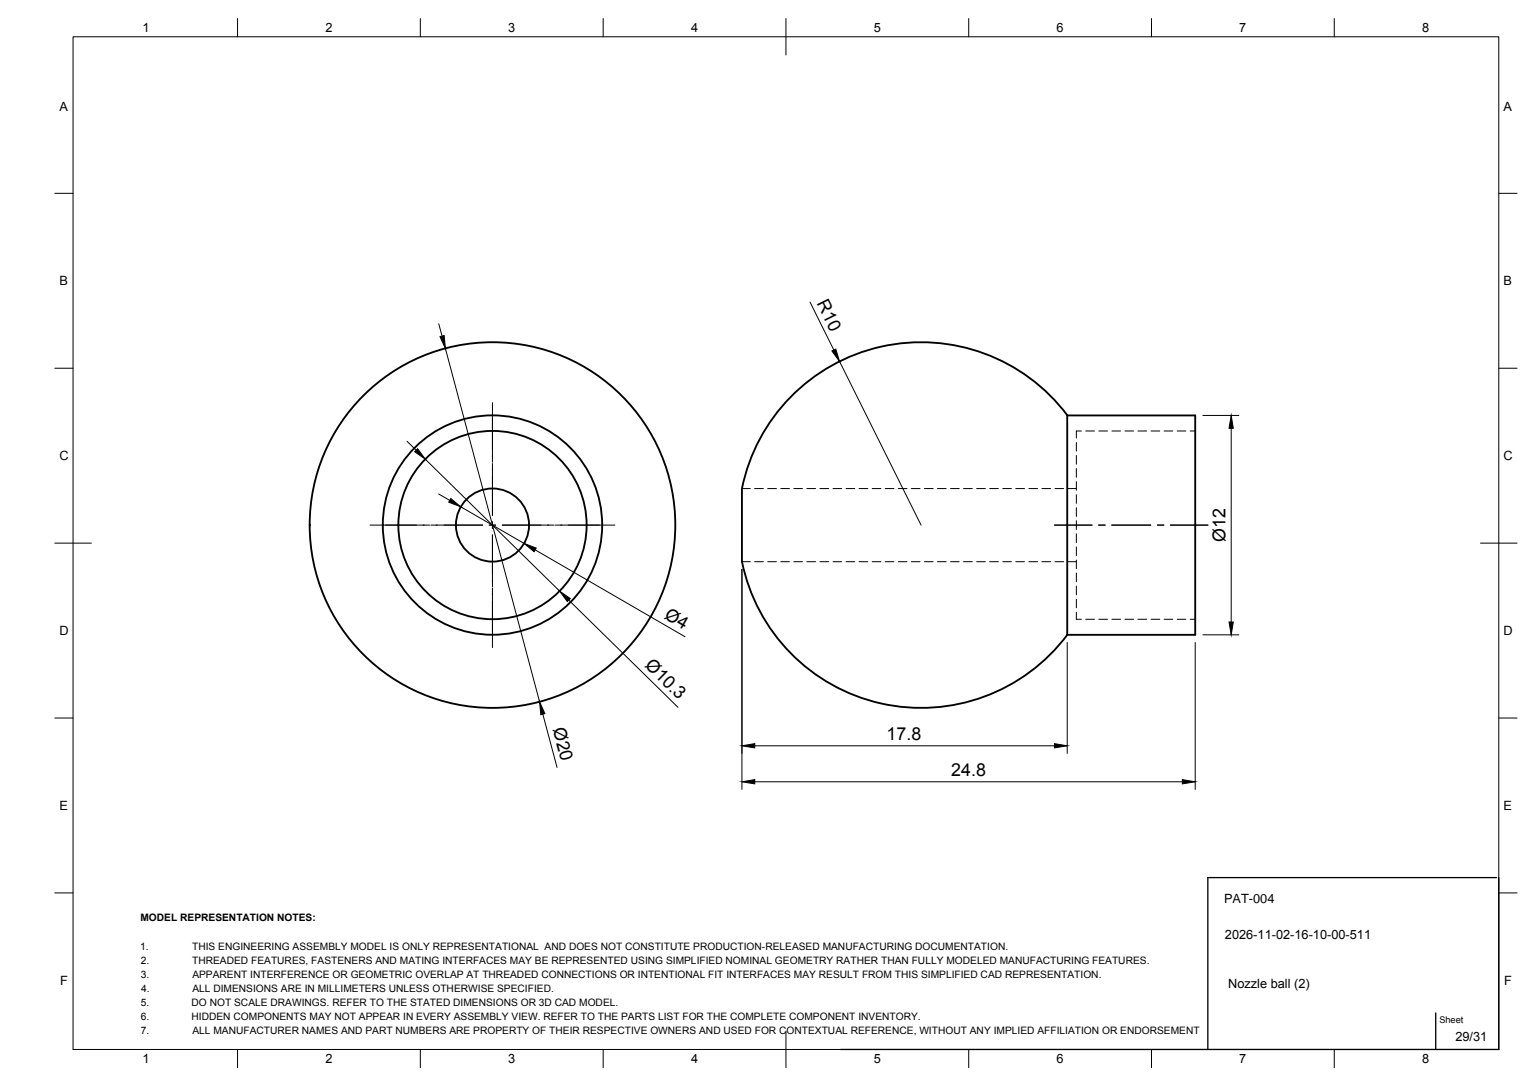
ISO-10303-21;
HEADER;
/* Generated by software containing ST-Developer
 * from STEP Tools, Inc. (www.steptools.com) 
 */

FILE_DESCRIPTION(
/* description */ ('Air blow-off nozzle station'),
/* implementation_level */ '2;1');

FILE_NAME(
/* name */ 'Nozzle ball (2).step',
/* time_stamp */ '2026-10-27T10:53:54-07:00',
/* author */ (''),
/* organization */ (''),
/* preprocessor_version */ 'ST-DEVELOPER v20.2',
/* originating_system */ 'Autodesk Translation Framework v15.17.0.0',
/* authorisation */ '');

FILE_SCHEMA (('AUTOMOTIVE_DESIGN { 1 0 10303 214 3 1 1 }'));
ENDSEC;

DATA;
#10=MECHANICAL_DESIGN_GEOMETRIC_PRESENTATION_REPRESENTATION('',(#257),#7897);
#170=SPHERICAL_SURFACE('',#4988,1.);
#207=SHAPE_REPRESENTATION_RELATIONSHIP('SRR','None',#8024,#232);
#232=ADVANCED_BREP_SHAPE_REPRESENTATION('',(#280),#7891);
#257=STYLED_ITEM('',(#8234),#280);
#280=MANIFOLD_SOLID_BREP('Body1',#4308);
#353=FACE_BOUND('',#1083,.T.);
#354=FACE_BOUND('',#1087,.T.);
#355=FACE_BOUND('',#1089,.T.);
#356=FACE_BOUND('',#1090,.T.);
#518=PLANE('',#4980);
#519=PLANE('',#4987);
#757=FACE_OUTER_BOUND('',#1081,.T.);
#758=FACE_OUTER_BOUND('',#1082,.T.);
#759=FACE_OUTER_BOUND('',#1084,.T.);
#760=FACE_OUTER_BOUND('',#1085,.T.);
#761=FACE_OUTER_BOUND('',#1086,.T.);
#762=FACE_OUTER_BOUND('',#1088,.T.);
#1081=EDGE_LOOP('',(#3825,#3826,#3827,#3828));
#1082=EDGE_LOOP('',(#3829));
#1083=EDGE_LOOP('',(#3830));
#1084=EDGE_LOOP('',(#3831,#3832,#3833,#3834));
#1085=EDGE_LOOP('',(#3835,#3836,#3837,#3838));
#1086=EDGE_LOOP('',(#3839));
#1087=EDGE_LOOP('',(#3840));
#1088=EDGE_LOOP('',(#3841,#3842));
#1089=EDGE_LOOP('',(#3843));
#1090=EDGE_LOOP('',(#3844));
#1458=LINE('',#7663,#1812);
#1459=LINE('',#7670,#1813);
#1460=LINE('',#7676,#1814);
#1812=VECTOR('',#6172,0.515);
#1813=VECTOR('',#6181,0.2);
#1814=VECTOR('',#6188,0.6);
#1974=CIRCLE('',#4978,0.515);
#1975=CIRCLE('',#4979,0.515);
#1976=CIRCLE('',#4981,0.2);
#1977=CIRCLE('',#4983,0.2);
#1978=CIRCLE('',#4985,0.6);
#1979=CIRCLE('',#4986,0.6);
#1980=CIRCLE('',#4989,1.);
#2320=VERTEX_POINT('',#7660);
#2321=VERTEX_POINT('',#7662);
#2322=VERTEX_POINT('',#7666);
#2323=VERTEX_POINT('',#7669);
#2324=VERTEX_POINT('',#7673);
#2325=VERTEX_POINT('',#7675);
#2326=VERTEX_POINT('',#7680);
#2327=VERTEX_POINT('',#7681);
#2830=EDGE_CURVE('',#2320,#2320,#1974,.T.);
#2831=EDGE_CURVE('',#2320,#2321,#1458,.T.);
#2832=EDGE_CURVE('',#2321,#2321,#1975,.T.);
#2833=EDGE_CURVE('',#2322,#2322,#1976,.T.);
#2834=EDGE_CURVE('',#2322,#2323,#1459,.T.);
#2835=EDGE_CURVE('',#2323,#2323,#1977,.T.);
#2836=EDGE_CURVE('',#2324,#2324,#1978,.T.);
#2837=EDGE_CURVE('',#2324,#2325,#1460,.T.);
#2838=EDGE_CURVE('',#2325,#2325,#1979,.T.);
#2839=EDGE_CURVE('',#2326,#2327,#1980,.T.);
#3825=ORIENTED_EDGE('',*,*,#2830,.F.);
#3826=ORIENTED_EDGE('',*,*,#2831,.T.);
#3827=ORIENTED_EDGE('',*,*,#2832,.T.);
#3828=ORIENTED_EDGE('',*,*,#2831,.F.);
#3829=ORIENTED_EDGE('',*,*,#2832,.F.);
#3830=ORIENTED_EDGE('',*,*,#2833,.F.);
#3831=ORIENTED_EDGE('',*,*,#2833,.T.);
#3832=ORIENTED_EDGE('',*,*,#2834,.T.);
#3833=ORIENTED_EDGE('',*,*,#2835,.F.);
#3834=ORIENTED_EDGE('',*,*,#2834,.F.);
#3835=ORIENTED_EDGE('',*,*,#2836,.F.);
#3836=ORIENTED_EDGE('',*,*,#2837,.T.);
#3837=ORIENTED_EDGE('',*,*,#2838,.T.);
#3838=ORIENTED_EDGE('',*,*,#2837,.F.);
#3839=ORIENTED_EDGE('',*,*,#2838,.F.);
#3840=ORIENTED_EDGE('',*,*,#2830,.T.);
#3841=ORIENTED_EDGE('',*,*,#2839,.T.);
#3842=ORIENTED_EDGE('',*,*,#2839,.F.);
#3843=ORIENTED_EDGE('',*,*,#2835,.T.);
#3844=ORIENTED_EDGE('',*,*,#2836,.T.);
#4014=CYLINDRICAL_SURFACE('',#4977,0.515);
#4015=CYLINDRICAL_SURFACE('',#4982,0.2);
#4016=CYLINDRICAL_SURFACE('',#4984,0.6);
#4247=ADVANCED_FACE('',(#757),#4014,.F.);
#4248=ADVANCED_FACE('',(#758,#353),#518,.F.);
#4249=ADVANCED_FACE('',(#759),#4015,.F.);
#4250=ADVANCED_FACE('',(#760),#4016,.T.);
#4251=ADVANCED_FACE('',(#761,#354),#519,.F.);
#4252=ADVANCED_FACE('',(#762,#355,#356),#170,.T.);
#4308=CLOSED_SHELL('',(#4247,#4248,#4249,#4250,#4251,#4252));
#4976=AXIS2_PLACEMENT_3D('',#7658,#6166,#6167);
#4977=AXIS2_PLACEMENT_3D('',#7659,#6168,#6169);
#4978=AXIS2_PLACEMENT_3D('',#7661,#6170,#6171);
#4979=AXIS2_PLACEMENT_3D('',#7664,#6173,#6174);
#4980=AXIS2_PLACEMENT_3D('',#7665,#6175,#6176);
#4981=AXIS2_PLACEMENT_3D('',#7667,#6177,#6178);
#4982=AXIS2_PLACEMENT_3D('',#7668,#6179,#6180);
#4983=AXIS2_PLACEMENT_3D('',#7671,#6182,#6183);
#4984=AXIS2_PLACEMENT_3D('',#7672,#6184,#6185);
#4985=AXIS2_PLACEMENT_3D('',#7674,#6186,#6187);
#4986=AXIS2_PLACEMENT_3D('',#7677,#6189,#6190);
#4987=AXIS2_PLACEMENT_3D('',#7678,#6191,#6192);
#4988=AXIS2_PLACEMENT_3D('',#7679,#6193,#6194);
#4989=AXIS2_PLACEMENT_3D('',#7682,#6195,#6196);
#6166=DIRECTION('axis',(0.,0.,1.));
#6167=DIRECTION('refdir',(1.,0.,0.));
#6168=DIRECTION('center_axis',(0.,1.,0.));
#6169=DIRECTION('ref_axis',(1.,0.,0.));
#6170=DIRECTION('center_axis',(0.,1.,0.));
#6171=DIRECTION('ref_axis',(1.,0.,0.));
#6172=DIRECTION('',(0.,1.,0.));
#6173=DIRECTION('center_axis',(0.,1.,0.));
#6174=DIRECTION('ref_axis',(1.,0.,0.));
#6175=DIRECTION('center_axis',(0.,1.,0.));
#6176=DIRECTION('ref_axis',(1.,0.,0.));
#6177=DIRECTION('center_axis',(0.,-1.,0.));
#6178=DIRECTION('ref_axis',(1.,0.,0.));
#6179=DIRECTION('center_axis',(0.,1.,0.));
#6180=DIRECTION('ref_axis',(1.,0.,0.));
#6181=DIRECTION('',(0.,1.,0.));
#6182=DIRECTION('center_axis',(0.,-1.,0.));
#6183=DIRECTION('ref_axis',(1.,-1.11022302462516E-15,0.));
#6184=DIRECTION('center_axis',(0.,1.,0.));
#6185=DIRECTION('ref_axis',(1.,0.,0.));
#6186=DIRECTION('center_axis',(0.,1.,0.));
#6187=DIRECTION('ref_axis',(1.,0.,0.));
#6188=DIRECTION('',(0.,-1.,0.));
#6189=DIRECTION('center_axis',(0.,1.,0.));
#6190=DIRECTION('ref_axis',(1.,0.,0.));
#6191=DIRECTION('center_axis',(0.,1.,0.));
#6192=DIRECTION('ref_axis',(1.,0.,0.));
#6193=DIRECTION('center_axis',(0.,0.,1.));
#6194=DIRECTION('ref_axis',(1.,0.,0.));
#6195=DIRECTION('center_axis',(0.,-1.,0.));
#6196=DIRECTION('ref_axis',(-1.,0.,0.));
#7658=CARTESIAN_POINT('',(0.,0.,0.));
#7659=CARTESIAN_POINT('Origin',(3.,-3.6,23.));
#7660=CARTESIAN_POINT('',(2.485,-3.5,23.));
#7661=CARTESIAN_POINT('Origin',(3.,-3.5,23.));
#7662=CARTESIAN_POINT('',(2.485,-2.85,23.));
#7663=CARTESIAN_POINT('',(2.485,-3.6,23.));
#7664=CARTESIAN_POINT('Origin',(3.,-2.85,23.));
#7665=CARTESIAN_POINT('Origin',(3.,-2.85,23.));
#7666=CARTESIAN_POINT('',(2.8,-2.85,23.));
#7667=CARTESIAN_POINT('Origin',(3.,-2.85,23.));
#7668=CARTESIAN_POINT('Origin',(3.,-3.6,23.));
#7669=CARTESIAN_POINT('',(2.8,-1.02020410288673,23.));
#7670=CARTESIAN_POINT('',(2.8,-3.6,23.));
#7671=CARTESIAN_POINT('Origin',(3.,-1.02020410288673,23.));
#7672=CARTESIAN_POINT('Origin',(3.,-3.5,23.));
#7673=CARTESIAN_POINT('',(2.4,-2.8,23.));
#7674=CARTESIAN_POINT('Origin',(3.,-2.8,23.));
#7675=CARTESIAN_POINT('',(2.4,-3.5,23.));
#7676=CARTESIAN_POINT('',(2.4,-3.5,23.));
#7677=CARTESIAN_POINT('Origin',(3.,-3.5,23.));
#7678=CARTESIAN_POINT('Origin',(3.,-3.5,23.));
#7679=CARTESIAN_POINT('Origin',(3.,-2.,23.));
#7680=CARTESIAN_POINT('',(3.,-2.,24.));
#7681=CARTESIAN_POINT('',(3.,-2.,22.));
#7682=CARTESIAN_POINT('Origin',(3.,-2.,23.));
#7859=UNCERTAINTY_MEASURE_WITH_UNIT(LENGTH_MEASURE(0.001),#7898,
'DISTANCE_ACCURACY_VALUE',
'Maximum model space distance between geometric entities at asserted c
onnectivities');
#7865=UNCERTAINTY_MEASURE_WITH_UNIT(LENGTH_MEASURE(0.001),#7898,
'DISTANCE_ACCURACY_VALUE',
'Maximum model space distance between geometric entities at asserted c
onnectivities');
#7891=(
GEOMETRIC_REPRESENTATION_CONTEXT(3)
GLOBAL_UNCERTAINTY_ASSIGNED_CONTEXT((#7859))
GLOBAL_UNIT_ASSIGNED_CONTEXT((#7898,#7900,#7901))
REPRESENTATION_CONTEXT('','3D')
);
#7897=(
GEOMETRIC_REPRESENTATION_CONTEXT(3)
GLOBAL_UNCERTAINTY_ASSIGNED_CONTEXT((#7865))
GLOBAL_UNIT_ASSIGNED_CONTEXT((#7898,#7900,#7901))
REPRESENTATION_CONTEXT('','3D')
);
#7898=(
LENGTH_UNIT()
NAMED_UNIT(*)
SI_UNIT(.CENTI.,.METRE.)
);
#7900=(
NAMED_UNIT(*)
PLANE_ANGLE_UNIT()
SI_UNIT($,.RADIAN.)
);
#7901=(
NAMED_UNIT(*)
SI_UNIT($,.STERADIAN.)
SOLID_ANGLE_UNIT()
);
#7927=SHAPE_DEFINITION_REPRESENTATION(#7975,#8024);
#7975=PRODUCT_DEFINITION_SHAPE('',$,#8056);
#8024=SHAPE_REPRESENTATION('',(#4976),#7891);
#8030=PRODUCT_DEFINITION_CONTEXT('part definition',#8125,'design');
#8056=PRODUCT_DEFINITION('Nozzle ball (2)','Nozzle ball (2)',#8087,#8030);
#8087=PRODUCT_DEFINITION_FORMATION('',$,#8152);
#8125=APPLICATION_CONTEXT(
'Core Data for Automotive Mechanical Design Process');
#8126=PRODUCT_CONTEXT('part definition',#8125,'mechanical');
#8152=PRODUCT('Nozzle ball (2)','Nozzle ball (2)','Nozzle ball (2)',(#8126));
#8228=COLOUR_RGB('Off White',0.89,0.88,0.83);
#8229=FILL_AREA_STYLE_COLOUR('',#8228);
#8230=FILL_AREA_STYLE('',(#8229));
#8231=SURFACE_STYLE_FILL_AREA(#8230);
#8232=SURFACE_SIDE_STYLE('',(#8231));
#8233=SURFACE_STYLE_USAGE(.BOTH.,#8232);
#8234=PRESENTATION_STYLE_ASSIGNMENT((#8233));
ENDSEC;
END-ISO-10303-21;
